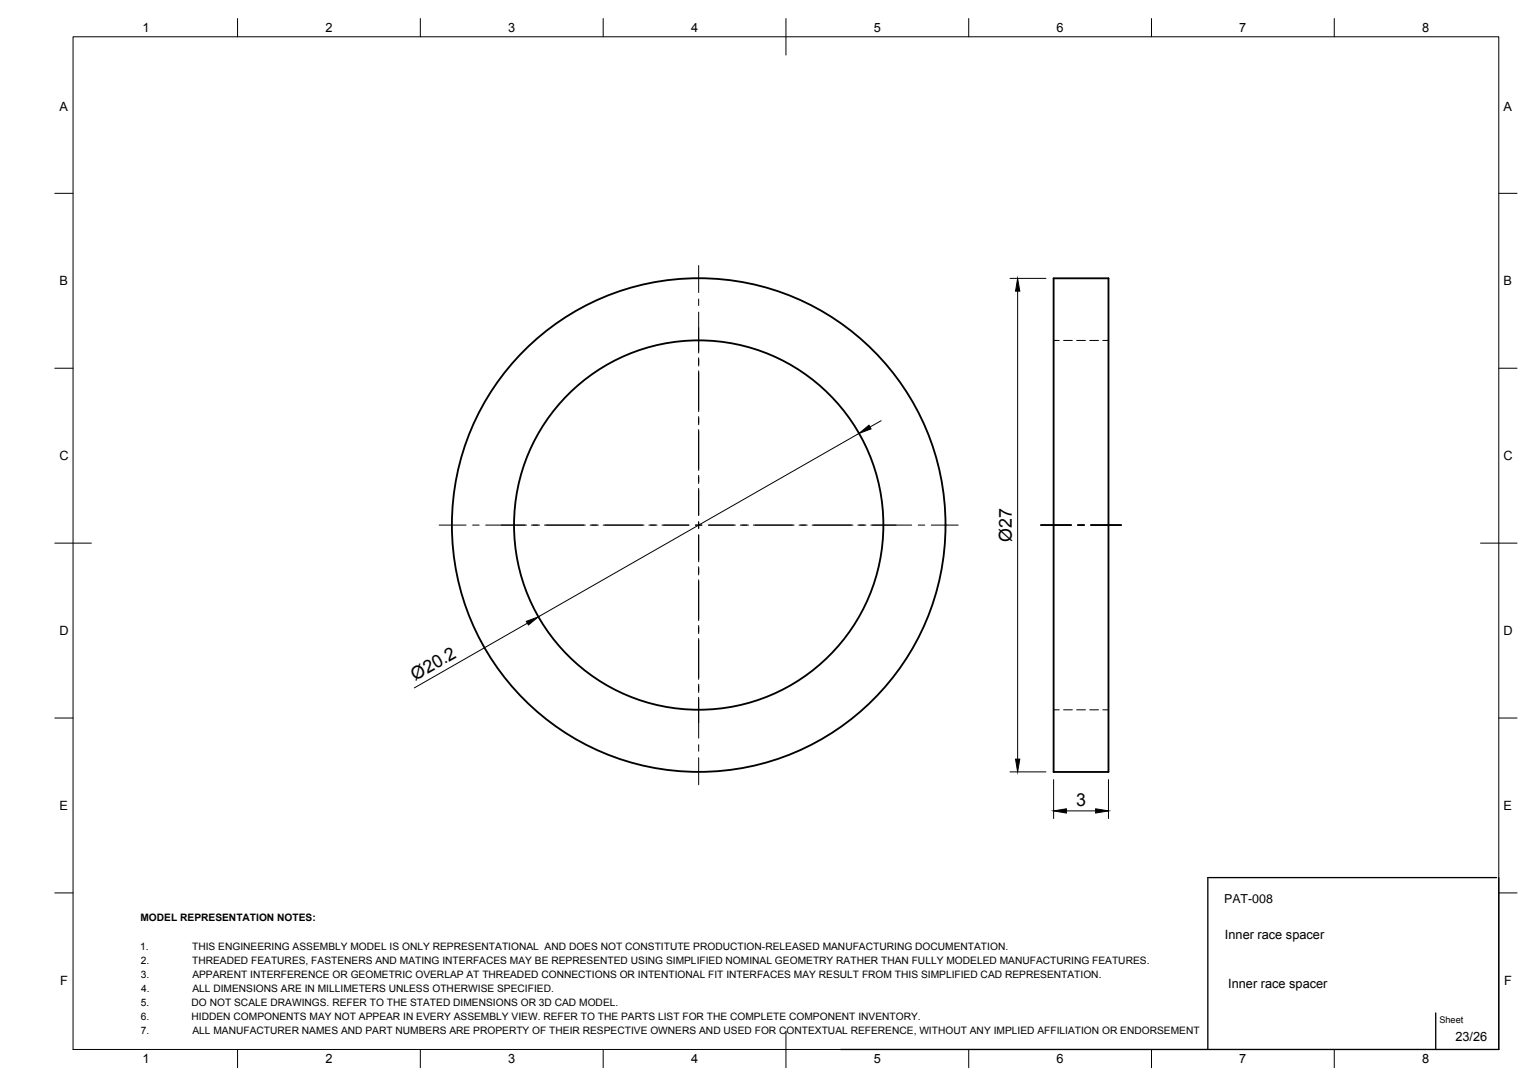
ISO-10303-21;
HEADER;
/* Generated by software containing ST-Developer
 * from STEP Tools, Inc. (www.steptools.com) 
 */

FILE_DESCRIPTION(
/* description */ ('Bearing housing with oil seal and end cap'),
/* implementation_level */ '2;1');

FILE_NAME(
/* name */ 'Inner race spacer.step',
/* time_stamp */ '2026-10-28T03:23:10-07:00',
/* author */ (''),
/* organization */ (''),
/* preprocessor_version */ 'ST-DEVELOPER v20.2',
/* originating_system */ 'Autodesk Translation Framework v15.17.0.0',
/* authorisation */ '');

FILE_SCHEMA (('AUTOMOTIVE_DESIGN { 1 0 10303 214 3 1 1 }'));
ENDSEC;

DATA;
#10=MECHANICAL_DESIGN_GEOMETRIC_PRESENTATION_REPRESENTATION('',(#283),#7871);
#233=SHAPE_REPRESENTATION_RELATIONSHIP('SRR','None',#7982,#254);
#254=ADVANCED_BREP_SHAPE_REPRESENTATION('',(#310),#7866);
#283=STYLED_ITEM('',(#8153),#310);
#310=MANIFOLD_SOLID_BREP('Body1',#4111);
#388=FACE_BOUND('',#1081,.T.);
#389=FACE_BOUND('',#1083,.T.);
#519=PLANE('',#4792);
#520=PLANE('',#4793);
#754=FACE_OUTER_BOUND('',#1078,.T.);
#755=FACE_OUTER_BOUND('',#1079,.T.);
#756=FACE_OUTER_BOUND('',#1080,.T.);
#757=FACE_OUTER_BOUND('',#1082,.T.);
#1078=EDGE_LOOP('',(#3537,#3538,#3539,#3540));
#1079=EDGE_LOOP('',(#3541,#3542,#3543,#3544));
#1080=EDGE_LOOP('',(#3545));
#1081=EDGE_LOOP('',(#3546));
#1082=EDGE_LOOP('',(#3547));
#1083=EDGE_LOOP('',(#3548));
#1338=LINE('',#7465,#1600);
#1339=LINE('',#7471,#1601);
#1600=VECTOR('',#5951,1.01);
#1601=VECTOR('',#5958,1.35);
#1859=CIRCLE('',#4787,1.01);
#1860=CIRCLE('',#4788,1.01);
#1861=CIRCLE('',#4790,1.35);
#1862=CIRCLE('',#4791,1.35);
#2161=VERTEX_POINT('',#7462);
#2162=VERTEX_POINT('',#7464);
#2163=VERTEX_POINT('',#7468);
#2164=VERTEX_POINT('',#7470);
#2632=EDGE_CURVE('',#2161,#2161,#1859,.T.);
#2633=EDGE_CURVE('',#2161,#2162,#1338,.T.);
#2634=EDGE_CURVE('',#2162,#2162,#1860,.T.);
#2635=EDGE_CURVE('',#2163,#2163,#1861,.T.);
#2636=EDGE_CURVE('',#2163,#2164,#1339,.T.);
#2637=EDGE_CURVE('',#2164,#2164,#1862,.T.);
#3537=ORIENTED_EDGE('',*,*,#2632,.F.);
#3538=ORIENTED_EDGE('',*,*,#2633,.T.);
#3539=ORIENTED_EDGE('',*,*,#2634,.T.);
#3540=ORIENTED_EDGE('',*,*,#2633,.F.);
#3541=ORIENTED_EDGE('',*,*,#2635,.F.);
#3542=ORIENTED_EDGE('',*,*,#2636,.T.);
#3543=ORIENTED_EDGE('',*,*,#2637,.T.);
#3544=ORIENTED_EDGE('',*,*,#2636,.F.);
#3545=ORIENTED_EDGE('',*,*,#2635,.T.);
#3546=ORIENTED_EDGE('',*,*,#2632,.T.);
#3547=ORIENTED_EDGE('',*,*,#2637,.F.);
#3548=ORIENTED_EDGE('',*,*,#2634,.F.);
#3820=CYLINDRICAL_SURFACE('',#4786,1.01);
#3821=CYLINDRICAL_SURFACE('',#4789,1.35);
#4036=ADVANCED_FACE('',(#754),#3820,.F.);
#4037=ADVANCED_FACE('',(#755),#3821,.T.);
#4038=ADVANCED_FACE('',(#756,#388),#519,.T.);
#4039=ADVANCED_FACE('',(#757,#389),#520,.F.);
#4111=CLOSED_SHELL('',(#4036,#4037,#4038,#4039));
#4785=AXIS2_PLACEMENT_3D('',#7460,#5945,#5946);
#4786=AXIS2_PLACEMENT_3D('',#7461,#5947,#5948);
#4787=AXIS2_PLACEMENT_3D('',#7463,#5949,#5950);
#4788=AXIS2_PLACEMENT_3D('',#7466,#5952,#5953);
#4789=AXIS2_PLACEMENT_3D('',#7467,#5954,#5955);
#4790=AXIS2_PLACEMENT_3D('',#7469,#5956,#5957);
#4791=AXIS2_PLACEMENT_3D('',#7472,#5959,#5960);
#4792=AXIS2_PLACEMENT_3D('',#7473,#5961,#5962);
#4793=AXIS2_PLACEMENT_3D('',#7474,#5963,#5964);
#5945=DIRECTION('axis',(0.,0.,1.));
#5946=DIRECTION('refdir',(1.,0.,0.));
#5947=DIRECTION('center_axis',(0.,1.,0.));
#5948=DIRECTION('ref_axis',(1.,0.,0.));
#5949=DIRECTION('center_axis',(0.,-1.,0.));
#5950=DIRECTION('ref_axis',(1.,0.,0.));
#5951=DIRECTION('',(0.,-1.,0.));
#5952=DIRECTION('center_axis',(0.,-1.,0.));
#5953=DIRECTION('ref_axis',(1.,0.,0.));
#5954=DIRECTION('center_axis',(0.,1.,0.));
#5955=DIRECTION('ref_axis',(1.,0.,0.));
#5956=DIRECTION('center_axis',(0.,1.,0.));
#5957=DIRECTION('ref_axis',(1.,0.,0.));
#5958=DIRECTION('',(0.,-1.,0.));
#5959=DIRECTION('center_axis',(0.,1.,0.));
#5960=DIRECTION('ref_axis',(1.,0.,0.));
#5961=DIRECTION('center_axis',(0.,1.,0.));
#5962=DIRECTION('ref_axis',(1.,0.,0.));
#5963=DIRECTION('center_axis',(0.,1.,0.));
#5964=DIRECTION('ref_axis',(1.,0.,0.));
#7460=CARTESIAN_POINT('',(0.,0.,0.));
#7461=CARTESIAN_POINT('Origin',(0.,5.7,4.5));
#7462=CARTESIAN_POINT('',(-1.01,6.,4.5));
#7463=CARTESIAN_POINT('Origin',(0.,6.,4.5));
#7464=CARTESIAN_POINT('',(-1.01,5.7,4.5));
#7465=CARTESIAN_POINT('',(-1.01,5.7,4.5));
#7466=CARTESIAN_POINT('Origin',(0.,5.7,4.5));
#7467=CARTESIAN_POINT('Origin',(0.,5.7,4.5));
#7468=CARTESIAN_POINT('',(-1.35,6.,4.5));
#7469=CARTESIAN_POINT('Origin',(0.,6.,4.5));
#7470=CARTESIAN_POINT('',(-1.35,5.7,4.5));
#7471=CARTESIAN_POINT('',(-1.35,5.7,4.5));
#7472=CARTESIAN_POINT('Origin',(0.,5.7,4.5));
#7473=CARTESIAN_POINT('Origin',(0.,6.,4.5));
#7474=CARTESIAN_POINT('Origin',(0.,5.7,4.5));
#7840=UNCERTAINTY_MEASURE_WITH_UNIT(LENGTH_MEASURE(0.001),#7872,
'DISTANCE_ACCURACY_VALUE',
'Maximum model space distance between geometric entities at asserted c
onnectivities');
#7845=UNCERTAINTY_MEASURE_WITH_UNIT(LENGTH_MEASURE(0.001),#7872,
'DISTANCE_ACCURACY_VALUE',
'Maximum model space distance between geometric entities at asserted c
onnectivities');
#7866=(
GEOMETRIC_REPRESENTATION_CONTEXT(3)
GLOBAL_UNCERTAINTY_ASSIGNED_CONTEXT((#7840))
GLOBAL_UNIT_ASSIGNED_CONTEXT((#7872,#7874,#7875))
REPRESENTATION_CONTEXT('','3D')
);
#7871=(
GEOMETRIC_REPRESENTATION_CONTEXT(3)
GLOBAL_UNCERTAINTY_ASSIGNED_CONTEXT((#7845))
GLOBAL_UNIT_ASSIGNED_CONTEXT((#7872,#7874,#7875))
REPRESENTATION_CONTEXT('','3D')
);
#7872=(
LENGTH_UNIT()
NAMED_UNIT(*)
SI_UNIT(.CENTI.,.METRE.)
);
#7874=(
NAMED_UNIT(*)
PLANE_ANGLE_UNIT()
SI_UNIT($,.RADIAN.)
);
#7875=(
NAMED_UNIT(*)
SI_UNIT($,.STERADIAN.)
SOLID_ANGLE_UNIT()
);
#7896=SHAPE_DEFINITION_REPRESENTATION(#7948,#7982);
#7948=PRODUCT_DEFINITION_SHAPE('',$,#8008);
#7982=SHAPE_REPRESENTATION('',(#4785),#7866);
#7987=PRODUCT_DEFINITION_CONTEXT('part definition',#8064,'design');
#8008=PRODUCT_DEFINITION('Inner race spacer','Inner race spacer',#8033,
#7987);
#8033=PRODUCT_DEFINITION_FORMATION('',$,#8086);
#8064=APPLICATION_CONTEXT(
'Core Data for Automotive Mechanical Design Process');
#8065=PRODUCT_CONTEXT('part definition',#8064,'mechanical');
#8086=PRODUCT('Inner race spacer','Inner race spacer',
'Inner race spacer',(#8065));
#8147=COLOUR_RGB('Grey',0.48,0.52,0.57);
#8148=FILL_AREA_STYLE_COLOUR('',#8147);
#8149=FILL_AREA_STYLE('',(#8148));
#8150=SURFACE_STYLE_FILL_AREA(#8149);
#8151=SURFACE_SIDE_STYLE('',(#8150));
#8152=SURFACE_STYLE_USAGE(.BOTH.,#8151);
#8153=PRESENTATION_STYLE_ASSIGNMENT((#8152));
ENDSEC;
END-ISO-10303-21;
